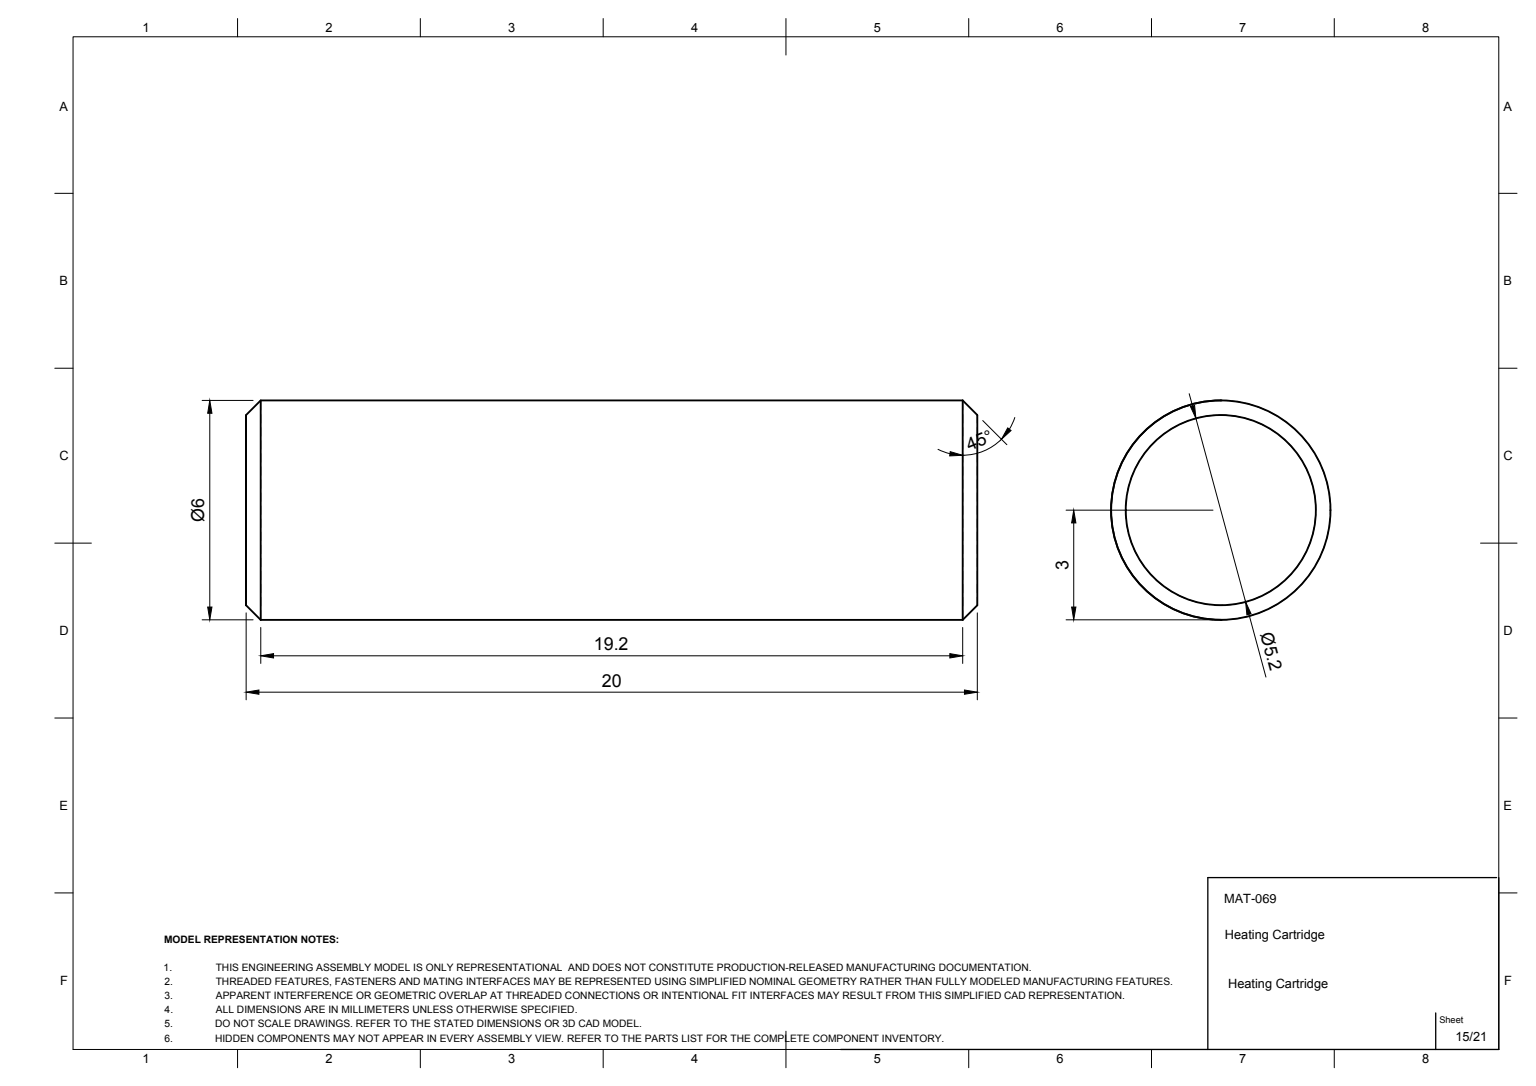
ISO-10303-21;
HEADER;
/* Generated by software containing ST-Developer
 * from STEP Tools, Inc. (www.steptools.com) 
 */

FILE_DESCRIPTION(
/* description */ ('CAx-IF Rec.Pracs.---Representation and Presentation of Product Manufa
cturing Information (PMI)---4.0---2014-10-13'),
/* implementation_level */ '2;1');

FILE_NAME(
/* name */ 'Heating Cartridge.step',
/* time_stamp */ '2026-10-24T15:08:39-07:00',
/* author */ (''),
/* organization */ (''),
/* preprocessor_version */ 'ST-DEVELOPER v20.2',
/* originating_system */ 'Autodesk Translation Framework v15.17.0.0',
/* authorisation */ '');

FILE_SCHEMA (('AP242_MANAGED_MODEL_BASED_3D_ENGINEERING_MIM_LF { 1 0 10303 442 2 1 4 }'));
ENDSEC;

DATA;
#10=MECHANICAL_DESIGN_GEOMETRIC_PRESENTATION_REPRESENTATION('',(#832),#50081);
#645=CONICAL_SURFACE('',#10670,0.0028,0.785398163397449);
#646=CONICAL_SURFACE('',#10676,0.0028,0.785398163397448);
#792=SHAPE_REPRESENTATION_RELATIONSHIP('SRR','None',#50160,#812);
#812=ADVANCED_BREP_SHAPE_REPRESENTATION('',(#852),#50073);
#832=STYLED_ITEM('',(#50258),#852);
#852=MANIFOLD_SOLID_BREP('Body1',#9877);
#1006=PLANE('',#10675);
#1007=PLANE('',#10678);
#1416=FACE_OUTER_BOUND('',#2000,.T.);
#1417=FACE_OUTER_BOUND('',#2001,.T.);
#1418=FACE_OUTER_BOUND('',#2002,.T.);
#1419=FACE_OUTER_BOUND('',#2003,.T.);
#1420=FACE_OUTER_BOUND('',#2004,.T.);
#2000=EDGE_LOOP('',(#7974,#7975,#7976,#7977));
#2001=EDGE_LOOP('',(#7978,#7979,#7980,#7981));
#2002=EDGE_LOOP('',(#7982));
#2003=EDGE_LOOP('',(#7983,#7984,#7985,#7986));
#2004=EDGE_LOOP('',(#7987));
#2533=LINE('',#40479,#3111);
#2534=LINE('',#40484,#3112);
#2535=LINE('',#40488,#3113);
#3111=VECTOR('',#12457,0.0028);
#3112=VECTOR('',#12464,0.003);
#3113=VECTOR('',#12469,0.0028);
#3628=CIRCLE('',#10671,0.00300000000001);
#3629=CIRCLE('',#10672,0.00260000000001);
#3630=CIRCLE('',#10674,0.00300000000001);
#3631=CIRCLE('',#10677,0.00260000000001);
#4383=VERTEX_POINT('',#40476);
#4384=VERTEX_POINT('',#40478);
#4385=VERTEX_POINT('',#40482);
#4386=VERTEX_POINT('',#40487);
#5640=EDGE_CURVE('',#4383,#4383,#3628,.T.);
#5641=EDGE_CURVE('',#4383,#4384,#2533,.T.);
#5642=EDGE_CURVE('',#4384,#4384,#3629,.T.);
#5643=EDGE_CURVE('',#4385,#4385,#3630,.T.);
#5644=EDGE_CURVE('',#4385,#4383,#2534,.T.);
#5645=EDGE_CURVE('',#4385,#4386,#2535,.T.);
#5646=EDGE_CURVE('',#4386,#4386,#3631,.T.);
#7974=ORIENTED_EDGE('',*,*,#5640,.T.);
#7975=ORIENTED_EDGE('',*,*,#5641,.T.);
#7976=ORIENTED_EDGE('',*,*,#5642,.T.);
#7977=ORIENTED_EDGE('',*,*,#5641,.F.);
#7978=ORIENTED_EDGE('',*,*,#5643,.F.);
#7979=ORIENTED_EDGE('',*,*,#5644,.T.);
#7980=ORIENTED_EDGE('',*,*,#5640,.F.);
#7981=ORIENTED_EDGE('',*,*,#5644,.F.);
#7982=ORIENTED_EDGE('',*,*,#5642,.F.);
#7983=ORIENTED_EDGE('',*,*,#5643,.T.);
#7984=ORIENTED_EDGE('',*,*,#5645,.T.);
#7985=ORIENTED_EDGE('',*,*,#5646,.T.);
#7986=ORIENTED_EDGE('',*,*,#5645,.F.);
#7987=ORIENTED_EDGE('',*,*,#5646,.F.);
#9250=CYLINDRICAL_SURFACE('',#10673,0.003);
#9638=ADVANCED_FACE('',(#1416),#645,.T.);
#9639=ADVANCED_FACE('',(#1417),#9250,.T.);
#9640=ADVANCED_FACE('',(#1418),#1006,.F.);
#9641=ADVANCED_FACE('',(#1419),#646,.T.);
#9642=ADVANCED_FACE('',(#1420),#1007,.T.);
#9877=CLOSED_SHELL('',(#9638,#9639,#9640,#9641,#9642));
#10669=AXIS2_PLACEMENT_3D('',#40474,#12451,#12452);
#10670=AXIS2_PLACEMENT_3D('',#40475,#12453,#12454);
#10671=AXIS2_PLACEMENT_3D('',#40477,#12455,#12456);
#10672=AXIS2_PLACEMENT_3D('',#40480,#12458,#12459);
#10673=AXIS2_PLACEMENT_3D('',#40481,#12460,#12461);
#10674=AXIS2_PLACEMENT_3D('',#40483,#12462,#12463);
#10675=AXIS2_PLACEMENT_3D('',#40485,#12465,#12466);
#10676=AXIS2_PLACEMENT_3D('',#40486,#12467,#12468);
#10677=AXIS2_PLACEMENT_3D('',#40489,#12470,#12471);
#10678=AXIS2_PLACEMENT_3D('',#40490,#12472,#12473);
#12451=DIRECTION('axis',(0.,0.,1.));
#12452=DIRECTION('refdir',(1.,0.,0.));
#12453=DIRECTION('center_axis',(-6.74488507274914E-15,1.49880108324396E-15,
-1.));
#12454=DIRECTION('ref_axis',(-0.173648177666927,-0.984807753012209,-3.04793925546002E-16));
#12455=DIRECTION('center_axis',(6.74488507274914E-15,-1.49880108324396E-15,
1.));
#12456=DIRECTION('ref_axis',(-0.173648177666927,-0.984807753012209,-3.04793925546002E-16));
#12457=DIRECTION('',(-0.122787803968966,-0.696364240320021,0.707106781186547));
#12458=DIRECTION('center_axis',(-6.74488507274914E-15,1.49880108324396E-15,
-1.));
#12459=DIRECTION('ref_axis',(-0.173648177666927,-0.984807753012209,-3.04793925546002E-16));
#12460=DIRECTION('center_axis',(-6.74488507274914E-15,1.49880108324396E-15,
-1.));
#12461=DIRECTION('ref_axis',(-0.173648177666927,-0.984807753012209,-3.04793925546002E-16));
#12462=DIRECTION('center_axis',(-6.74488507274914E-15,1.49880108324396E-15,
-1.));
#12463=DIRECTION('ref_axis',(-0.173648177666927,-0.984807753012209,-3.04793925546002E-16));
#12464=DIRECTION('',(6.74488507274914E-15,-1.49880108324396E-15,1.));
#12465=DIRECTION('center_axis',(-6.74488507274914E-15,1.49880108324396E-15,
-1.));
#12466=DIRECTION('ref_axis',(-0.173648177666927,-0.984807753012209,-3.04793925546002E-16));
#12467=DIRECTION('center_axis',(6.74488507274914E-15,-1.49880108324396E-15,
1.));
#12468=DIRECTION('ref_axis',(-0.173648177666927,-0.984807753012209,-3.04793925546002E-16));
#12469=DIRECTION('',(-0.122787803968975,-0.696364240320018,-0.707106781186548));
#12470=DIRECTION('center_axis',(6.74488507274914E-15,-1.49880108324396E-15,
1.));
#12471=DIRECTION('ref_axis',(-0.173648177666927,-0.984807753012209,-3.04793925546002E-16));
#12472=DIRECTION('center_axis',(-6.74488507274914E-15,1.49880108324396E-15,
-1.));
#12473=DIRECTION('ref_axis',(-0.173648177666927,-0.984807753012209,-3.04793925546002E-16));
#40474=CARTESIAN_POINT('',(0.,0.,0.));
#40475=CARTESIAN_POINT('Origin',(-0.0065,-0.0372787743898723,-0.00237585328655808));
#40476=CARTESIAN_POINT('',(-0.00597905546699748,-0.0343243511308258,-0.00257585328656808));
#40477=CARTESIAN_POINT('Origin',(-0.0065,-0.0372787743898723,-0.00257585328656808));
#40478=CARTESIAN_POINT('',(-0.00604851473806512,-0.0347182742320356,-0.00217585328656308));
#40479=CARTESIAN_POINT('',(-0.0060137851025326,-0.0345213126814381,-0.00237585328655808));
#40480=CARTESIAN_POINT('Origin',(-0.0065,-0.0372787743898723,-0.00217585328655808));
#40481=CARTESIAN_POINT('Origin',(-0.0065,-0.0372787743898723,-0.00217585328655808));
#40482=CARTESIAN_POINT('',(-0.00597905546699935,-0.0343243511308356,-0.0217758532865681));
#40483=CARTESIAN_POINT('Origin',(-0.00650000000000013,-0.0372787743898722,
-0.0217758532865681));
#40484=CARTESIAN_POINT('',(-0.00597905546699922,-0.0343243511308357,-0.00217585328655808));
#40485=CARTESIAN_POINT('Origin',(-0.0065,-0.0372787743898723,-0.00217585328655808));
#40486=CARTESIAN_POINT('Origin',(-0.00650000000000013,-0.0372787743898722,
-0.0219758532865581));
#40487=CARTESIAN_POINT('',(-0.00604851473806612,-0.0347182742320405,-0.0221758532865581));
#40488=CARTESIAN_POINT('',(-0.00601378510253273,-0.034521312681438,-0.0219758532865581));
#40489=CARTESIAN_POINT('Origin',(-0.00650000000000013,-0.0372787743898722,
-0.0221758532865681));
#40490=CARTESIAN_POINT('Origin',(-0.00650000000000013,-0.0372787743898722,
-0.0221758532865581));
#50051=UNCERTAINTY_MEASURE_WITH_UNIT(LENGTH_MEASURE(1.E-5),#50082,
'DISTANCE_ACCURACY_VALUE',
'Maximum model space distance between geometric entities at asserted c
onnectivities');
#50059=UNCERTAINTY_MEASURE_WITH_UNIT(LENGTH_MEASURE(1.E-5),#50082,
'DISTANCE_ACCURACY_VALUE',
'Maximum model space distance between geometric entities at asserted c
onnectivities');
#50073=(
GEOMETRIC_REPRESENTATION_CONTEXT(3)
GLOBAL_UNCERTAINTY_ASSIGNED_CONTEXT((#50051))
GLOBAL_UNIT_ASSIGNED_CONTEXT((#50082,#50083,#50084))
REPRESENTATION_CONTEXT('','3D')
);
#50081=(
GEOMETRIC_REPRESENTATION_CONTEXT(3)
GLOBAL_UNCERTAINTY_ASSIGNED_CONTEXT((#50059))
GLOBAL_UNIT_ASSIGNED_CONTEXT((#50082,#50083,#50084))
REPRESENTATION_CONTEXT('','3D')
);
#50082=(
LENGTH_UNIT()
NAMED_UNIT(*)
SI_UNIT($,.METRE.)
);
#50083=(
NAMED_UNIT(*)
PLANE_ANGLE_UNIT()
SI_UNIT($,.RADIAN.)
);
#50084=(
NAMED_UNIT(*)
SI_UNIT($,.STERADIAN.)
SOLID_ANGLE_UNIT()
);
#50098=SHAPE_DEFINITION_REPRESENTATION(#50119,#50160);
#50119=PRODUCT_DEFINITION_SHAPE('',$,#50182);
#50160=SHAPE_REPRESENTATION('',(#10669),#50073);
#50168=PRODUCT_DEFINITION_CONTEXT('part definition',#50233,'design');
#50182=PRODUCT_DEFINITION('Heating Cartridge','Heating Cartridge',#50203,
#50168);
#50203=PRODUCT_DEFINITION_FORMATION('',$,#50248);
#50233=APPLICATION_CONTEXT('Managed model based 3d engineering');
#50234=PRODUCT_CONTEXT('part definition',#50233,'mechanical');
#50248=PRODUCT('Heating Cartridge','Heating Cartridge',
'LEGAL AND USAGE DISCLAIMER: this Data/Model is provided \X2\201C\X0\A
S IS\X2\201D\X0\ for informational and representational only. It is a 
geometric approximation and is NOT engineered, certified, or guarantee
d for dimensional accuracy, exact tolerances, or production-level prec
ision. Vendor disclaims all implied warranties including fitness for a
 particular purpose. DO NOT USE FOR DIRECT PHYSICAL MANUFACTURING, AUT
OMATED PRODUCTION, OR SAFETY-CRITICAL SYSTEMS without independent engi
neering verification and resolution of any design discrepancies.',(#50234));
#50258=PRESENTATION_STYLE_ASSIGNMENT((#50265));
#50265=SURFACE_STYLE_USAGE(.BOTH.,#50272);
#50272=SURFACE_SIDE_STYLE('',(#50279));
#50279=SURFACE_STYLE_FILL_AREA(#50286);
#50286=FILL_AREA_STYLE('Opaque(89,149,218)',(#50293));
#50293=FILL_AREA_STYLE_COLOUR('Opaque(89,149,218)',#50300);
#50300=COLOUR_RGB('Opaque(89,149,218)',0.349019607843137,0.584313725490196,
0.854901960784314);
ENDSEC;
END-ISO-10303-21;
